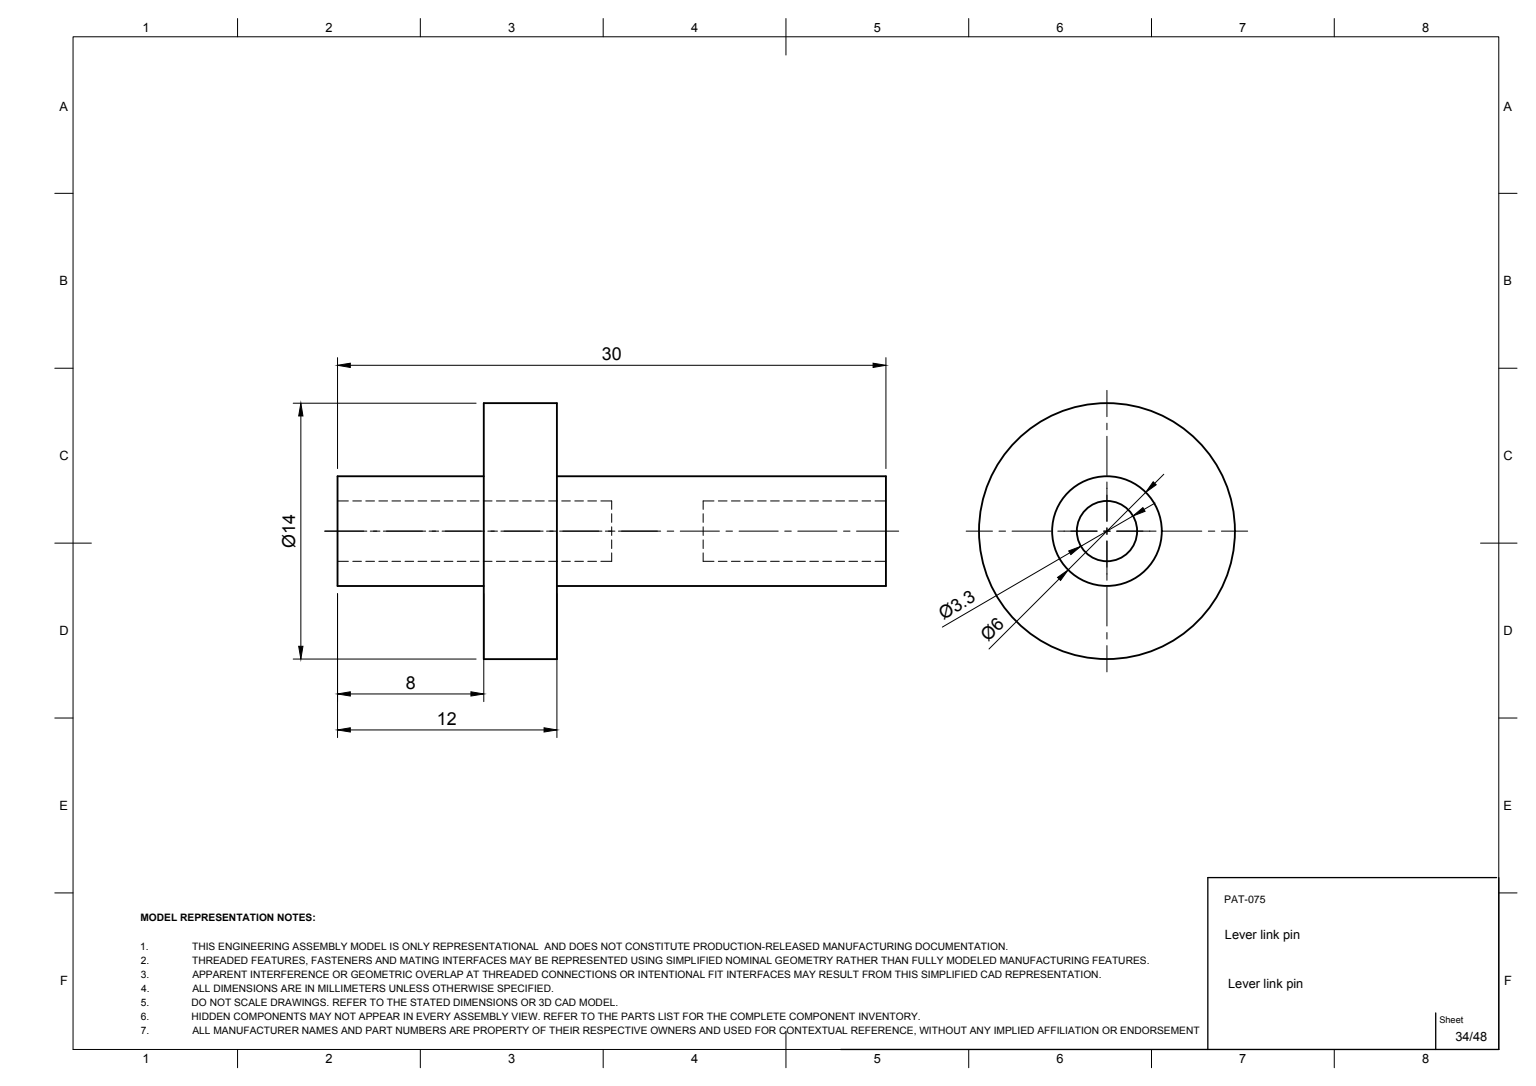
ISO-10303-21;
HEADER;
/* Generated by software containing ST-Developer
 * from STEP Tools, Inc. (www.steptools.com) 
 */

FILE_DESCRIPTION(
/* description */ ('Over-Centre Plunger Toggle Clamp on Slotted Fixture Frame'),
/* implementation_level */ '2;1');

FILE_NAME(
/* name */ 
'Lever link pin.step',
/* time_stamp */ '2026-10-28T03:23:24-07:00',
/* author */ (''),
/* organization */ (''),
/* preprocessor_version */ 'ST-DEVELOPER v20.2',
/* originating_system */ 'Autodesk Translation Framework v15.17.0.0',
/* authorisation */ '');

FILE_SCHEMA (('AUTOMOTIVE_DESIGN { 1 0 10303 214 3 1 1 }'));
ENDSEC;

DATA;
#10=MECHANICAL_DESIGN_GEOMETRIC_PRESENTATION_REPRESENTATION('',(#548),#15212);
#456=SHAPE_REPRESENTATION_RELATIONSHIP('SRR','None',#15433,#498);
#498=ADVANCED_BREP_SHAPE_REPRESENTATION('',(#597),#15195);
#548=STYLED_ITEM('',(#15719),#597);
#597=MANIFOLD_SOLID_BREP('Body1',#8282);
#753=FACE_BOUND('',#2075,.T.);
#754=FACE_BOUND('',#2077,.T.);
#755=FACE_BOUND('',#2082,.T.);
#756=FACE_BOUND('',#2084,.T.);
#1001=PLANE('',#9446);
#1002=PLANE('',#9450);
#1003=PLANE('',#9451);
#1004=PLANE('',#9454);
#1005=PLANE('',#9462);
#1006=PLANE('',#9463);
#1442=FACE_OUTER_BOUND('',#2070,.T.);
#1443=FACE_OUTER_BOUND('',#2071,.T.);
#1444=FACE_OUTER_BOUND('',#2072,.T.);
#1445=FACE_OUTER_BOUND('',#2073,.T.);
#1446=FACE_OUTER_BOUND('',#2074,.T.);
#1447=FACE_OUTER_BOUND('',#2076,.T.);
#1448=FACE_OUTER_BOUND('',#2078,.T.);
#1449=FACE_OUTER_BOUND('',#2079,.T.);
#1450=FACE_OUTER_BOUND('',#2080,.T.);
#1451=FACE_OUTER_BOUND('',#2081,.T.);
#1452=FACE_OUTER_BOUND('',#2083,.T.);
#2070=EDGE_LOOP('',(#7129,#7130,#7131,#7132));
#2071=EDGE_LOOP('',(#7133));
#2072=EDGE_LOOP('',(#7134,#7135,#7136,#7137));
#2073=EDGE_LOOP('',(#7138));
#2074=EDGE_LOOP('',(#7139));
#2075=EDGE_LOOP('',(#7140));
#2076=EDGE_LOOP('',(#7141));
#2077=EDGE_LOOP('',(#7142));
#2078=EDGE_LOOP('',(#7143,#7144,#7145,#7146));
#2079=EDGE_LOOP('',(#7147,#7148,#7149,#7150));
#2080=EDGE_LOOP('',(#7151,#7152,#7153,#7154));
#2081=EDGE_LOOP('',(#7155));
#2082=EDGE_LOOP('',(#7156));
#2083=EDGE_LOOP('',(#7157));
#2084=EDGE_LOOP('',(#7158));
#2704=LINE('',#14470,#3334);
#2705=LINE('',#14477,#3335);
#2706=LINE('',#14491,#3336);
#2707=LINE('',#14494,#3337);
#2708=LINE('',#14499,#3338);
#3334=VECTOR('',#11591,0.165);
#3335=VECTOR('',#11600,0.165);
#3336=VECTOR('',#11619,0.7);
#3337=VECTOR('',#11622,0.3);
#3338=VECTOR('',#11629,0.3);
#3774=CIRCLE('',#9444,0.165);
#3775=CIRCLE('',#9445,0.165);
#3776=CIRCLE('',#9448,0.165);
#3777=CIRCLE('',#9449,0.165);
#3778=CIRCLE('',#9452,0.7);
#3779=CIRCLE('',#9453,0.3);
#3780=CIRCLE('',#9455,0.7);
#3781=CIRCLE('',#9456,0.3);
#3782=CIRCLE('',#9459,0.3);
#3783=CIRCLE('',#9461,0.3);
#4386=VERTEX_POINT('',#14467);
#4387=VERTEX_POINT('',#14469);
#4388=VERTEX_POINT('',#14474);
#4389=VERTEX_POINT('',#14476);
#4390=VERTEX_POINT('',#14481);
#4391=VERTEX_POINT('',#14483);
#4392=VERTEX_POINT('',#14486);
#4393=VERTEX_POINT('',#14488);
#4394=VERTEX_POINT('',#14493);
#4395=VERTEX_POINT('',#14497);
#5325=EDGE_CURVE('',#4386,#4386,#3774,.T.);
#5326=EDGE_CURVE('',#4386,#4387,#2704,.T.);
#5327=EDGE_CURVE('',#4387,#4387,#3775,.T.);
#5328=EDGE_CURVE('',#4388,#4388,#3776,.T.);
#5329=EDGE_CURVE('',#4388,#4389,#2705,.T.);
#5330=EDGE_CURVE('',#4389,#4389,#3777,.T.);
#5331=EDGE_CURVE('',#4390,#4390,#3778,.T.);
#5332=EDGE_CURVE('',#4391,#4391,#3779,.T.);
#5333=EDGE_CURVE('',#4392,#4392,#3780,.T.);
#5334=EDGE_CURVE('',#4393,#4393,#3781,.T.);
#5335=EDGE_CURVE('',#4390,#4392,#2706,.T.);
#5336=EDGE_CURVE('',#4393,#4394,#2707,.T.);
#5337=EDGE_CURVE('',#4394,#4394,#3782,.T.);
#5338=EDGE_CURVE('',#4395,#4395,#3783,.T.);
#5339=EDGE_CURVE('',#4395,#4391,#2708,.T.);
#7129=ORIENTED_EDGE('',*,*,#5325,.F.);
#7130=ORIENTED_EDGE('',*,*,#5326,.T.);
#7131=ORIENTED_EDGE('',*,*,#5327,.F.);
#7132=ORIENTED_EDGE('',*,*,#5326,.F.);
#7133=ORIENTED_EDGE('',*,*,#5325,.T.);
#7134=ORIENTED_EDGE('',*,*,#5328,.F.);
#7135=ORIENTED_EDGE('',*,*,#5329,.T.);
#7136=ORIENTED_EDGE('',*,*,#5330,.T.);
#7137=ORIENTED_EDGE('',*,*,#5329,.F.);
#7138=ORIENTED_EDGE('',*,*,#5330,.F.);
#7139=ORIENTED_EDGE('',*,*,#5331,.T.);
#7140=ORIENTED_EDGE('',*,*,#5332,.F.);
#7141=ORIENTED_EDGE('',*,*,#5333,.F.);
#7142=ORIENTED_EDGE('',*,*,#5334,.F.);
#7143=ORIENTED_EDGE('',*,*,#5331,.F.);
#7144=ORIENTED_EDGE('',*,*,#5335,.T.);
#7145=ORIENTED_EDGE('',*,*,#5333,.T.);
#7146=ORIENTED_EDGE('',*,*,#5335,.F.);
#7147=ORIENTED_EDGE('',*,*,#5334,.T.);
#7148=ORIENTED_EDGE('',*,*,#5336,.T.);
#7149=ORIENTED_EDGE('',*,*,#5337,.T.);
#7150=ORIENTED_EDGE('',*,*,#5336,.F.);
#7151=ORIENTED_EDGE('',*,*,#5338,.F.);
#7152=ORIENTED_EDGE('',*,*,#5339,.T.);
#7153=ORIENTED_EDGE('',*,*,#5332,.T.);
#7154=ORIENTED_EDGE('',*,*,#5339,.F.);
#7155=ORIENTED_EDGE('',*,*,#5338,.T.);
#7156=ORIENTED_EDGE('',*,*,#5327,.T.);
#7157=ORIENTED_EDGE('',*,*,#5337,.F.);
#7158=ORIENTED_EDGE('',*,*,#5328,.T.);
#7724=CYLINDRICAL_SURFACE('',#9443,0.165);
#7725=CYLINDRICAL_SURFACE('',#9447,0.165);
#7726=CYLINDRICAL_SURFACE('',#9457,0.7);
#7727=CYLINDRICAL_SURFACE('',#9458,0.3);
#7728=CYLINDRICAL_SURFACE('',#9460,0.3);
#8114=ADVANCED_FACE('',(#1442),#7724,.F.);
#8115=ADVANCED_FACE('',(#1443),#1001,.T.);
#8116=ADVANCED_FACE('',(#1444),#7725,.F.);
#8117=ADVANCED_FACE('',(#1445),#1002,.F.);
#8118=ADVANCED_FACE('',(#1446,#753),#1003,.T.);
#8119=ADVANCED_FACE('',(#1447,#754),#1004,.F.);
#8120=ADVANCED_FACE('',(#1448),#7726,.T.);
#8121=ADVANCED_FACE('',(#1449),#7727,.T.);
#8122=ADVANCED_FACE('',(#1450),#7728,.T.);
#8123=ADVANCED_FACE('',(#1451,#755),#1005,.T.);
#8124=ADVANCED_FACE('',(#1452,#756),#1006,.F.);
#8282=CLOSED_SHELL('',(#8114,#8115,#8116,#8117,#8118,#8119,#8120,#8121,
#8122,#8123,#8124));
#9442=AXIS2_PLACEMENT_3D('',#14465,#11585,#11586);
#9443=AXIS2_PLACEMENT_3D('',#14466,#11587,#11588);
#9444=AXIS2_PLACEMENT_3D('',#14468,#11589,#11590);
#9445=AXIS2_PLACEMENT_3D('',#14471,#11592,#11593);
#9446=AXIS2_PLACEMENT_3D('',#14472,#11594,#11595);
#9447=AXIS2_PLACEMENT_3D('',#14473,#11596,#11597);
#9448=AXIS2_PLACEMENT_3D('',#14475,#11598,#11599);
#9449=AXIS2_PLACEMENT_3D('',#14478,#11601,#11602);
#9450=AXIS2_PLACEMENT_3D('',#14479,#11603,#11604);
#9451=AXIS2_PLACEMENT_3D('',#14480,#11605,#11606);
#9452=AXIS2_PLACEMENT_3D('',#14482,#11607,#11608);
#9453=AXIS2_PLACEMENT_3D('',#14484,#11609,#11610);
#9454=AXIS2_PLACEMENT_3D('',#14485,#11611,#11612);
#9455=AXIS2_PLACEMENT_3D('',#14487,#11613,#11614);
#9456=AXIS2_PLACEMENT_3D('',#14489,#11615,#11616);
#9457=AXIS2_PLACEMENT_3D('',#14490,#11617,#11618);
#9458=AXIS2_PLACEMENT_3D('',#14492,#11620,#11621);
#9459=AXIS2_PLACEMENT_3D('',#14495,#11623,#11624);
#9460=AXIS2_PLACEMENT_3D('',#14496,#11625,#11626);
#9461=AXIS2_PLACEMENT_3D('',#14498,#11627,#11628);
#9462=AXIS2_PLACEMENT_3D('',#14500,#11630,#11631);
#9463=AXIS2_PLACEMENT_3D('',#14501,#11632,#11633);
#11585=DIRECTION('axis',(0.,0.,1.));
#11586=DIRECTION('refdir',(1.,0.,0.));
#11587=DIRECTION('center_axis',(0.,1.,0.));
#11588=DIRECTION('ref_axis',(1.,0.,0.));
#11589=DIRECTION('center_axis',(0.,1.,0.));
#11590=DIRECTION('ref_axis',(1.,0.,0.));
#11591=DIRECTION('',(0.,1.,0.));
#11592=DIRECTION('center_axis',(0.,-1.,0.));
#11593=DIRECTION('ref_axis',(1.,0.,0.));
#11594=DIRECTION('center_axis',(0.,1.,0.));
#11595=DIRECTION('ref_axis',(1.,0.,0.));
#11596=DIRECTION('center_axis',(0.,1.,0.));
#11597=DIRECTION('ref_axis',(1.,0.,0.));
#11598=DIRECTION('center_axis',(0.,1.,0.));
#11599=DIRECTION('ref_axis',(1.,0.,0.));
#11600=DIRECTION('',(0.,1.,0.));
#11601=DIRECTION('center_axis',(0.,1.,0.));
#11602=DIRECTION('ref_axis',(1.,0.,0.));
#11603=DIRECTION('center_axis',(0.,1.,0.));
#11604=DIRECTION('ref_axis',(1.,0.,0.));
#11605=DIRECTION('center_axis',(0.,1.,0.));
#11606=DIRECTION('ref_axis',(1.,0.,0.));
#11607=DIRECTION('center_axis',(0.,1.,0.));
#11608=DIRECTION('ref_axis',(1.,0.,0.));
#11609=DIRECTION('center_axis',(0.,1.,0.));
#11610=DIRECTION('ref_axis',(1.,0.,0.));
#11611=DIRECTION('center_axis',(0.,1.,0.));
#11612=DIRECTION('ref_axis',(1.,0.,0.));
#11613=DIRECTION('center_axis',(0.,1.,0.));
#11614=DIRECTION('ref_axis',(1.,0.,0.));
#11615=DIRECTION('center_axis',(0.,-1.,0.));
#11616=DIRECTION('ref_axis',(1.,0.,0.));
#11617=DIRECTION('center_axis',(0.,1.,0.));
#11618=DIRECTION('ref_axis',(1.,0.,0.));
#11619=DIRECTION('',(0.,-1.,0.));
#11620=DIRECTION('center_axis',(0.,1.,0.));
#11621=DIRECTION('ref_axis',(1.,0.,0.));
#11622=DIRECTION('',(0.,-1.,0.));
#11623=DIRECTION('center_axis',(0.,1.,0.));
#11624=DIRECTION('ref_axis',(1.,0.,0.));
#11625=DIRECTION('center_axis',(0.,1.,0.));
#11626=DIRECTION('ref_axis',(1.,0.,0.));
#11627=DIRECTION('center_axis',(0.,1.,0.));
#11628=DIRECTION('ref_axis',(1.,0.,0.));
#11629=DIRECTION('',(0.,-1.,0.));
#11630=DIRECTION('center_axis',(0.,1.,0.));
#11631=DIRECTION('ref_axis',(1.,0.,0.));
#11632=DIRECTION('center_axis',(0.,1.,0.));
#11633=DIRECTION('ref_axis',(1.,0.,0.));
#14465=CARTESIAN_POINT('',(0.,0.,0.));
#14466=CARTESIAN_POINT('Origin',(-2.82632109303527,-4.2,8.79263101785268));
#14467=CARTESIAN_POINT('',(-2.99132109303527,-4.2,8.79263101785268));
#14468=CARTESIAN_POINT('Origin',(-2.82632109303527,-4.2,8.79263101785268));
#14469=CARTESIAN_POINT('',(-2.99132109303527,-2.7,8.79263101785268));
#14470=CARTESIAN_POINT('',(-2.99132109303527,-4.2,8.79263101785268));
#14471=CARTESIAN_POINT('Origin',(-2.82632109303527,-2.7,8.79263101785268));
#14472=CARTESIAN_POINT('Origin',(-2.82632109303527,-4.2,8.79263101785268));
#14473=CARTESIAN_POINT('Origin',(-2.82632109303527,-5.8,8.79263101785268));
#14474=CARTESIAN_POINT('',(-2.99132109303527,-5.7,8.79263101785268));
#14475=CARTESIAN_POINT('Origin',(-2.82632109303527,-5.7,8.79263101785268));
#14476=CARTESIAN_POINT('',(-2.99132109303527,-4.7,8.79263101785268));
#14477=CARTESIAN_POINT('',(-2.99132109303527,-5.8,8.79263101785268));
#14478=CARTESIAN_POINT('Origin',(-2.82632109303527,-4.7,8.79263101785268));
#14479=CARTESIAN_POINT('Origin',(-2.82632109303527,-4.7,8.79263101785268));
#14480=CARTESIAN_POINT('Origin',(-2.82632109303527,-3.5,8.79263101785268));
#14481=CARTESIAN_POINT('',(-3.52632109303527,-3.5,8.79263101785268));
#14482=CARTESIAN_POINT('Origin',(-2.82632109303527,-3.5,8.79263101785268));
#14483=CARTESIAN_POINT('',(-3.12632109303527,-3.5,8.79263101785268));
#14484=CARTESIAN_POINT('Origin',(-2.82632109303527,-3.5,8.79263101785268));
#14485=CARTESIAN_POINT('Origin',(-2.82632109303527,-3.9,8.79263101785268));
#14486=CARTESIAN_POINT('',(-3.52632109303527,-3.9,8.79263101785268));
#14487=CARTESIAN_POINT('Origin',(-2.82632109303527,-3.9,8.79263101785268));
#14488=CARTESIAN_POINT('',(-3.12632109303527,-3.9,8.79263101785268));
#14489=CARTESIAN_POINT('Origin',(-2.82632109303527,-3.9,8.79263101785268));
#14490=CARTESIAN_POINT('Origin',(-2.82632109303527,-3.9,8.79263101785268));
#14491=CARTESIAN_POINT('',(-3.52632109303527,-3.9,8.79263101785268));
#14492=CARTESIAN_POINT('Origin',(-2.82632109303527,-5.7,8.79263101785268));
#14493=CARTESIAN_POINT('',(-3.12632109303527,-5.7,8.79263101785268));
#14494=CARTESIAN_POINT('',(-3.12632109303527,-5.7,8.79263101785268));
#14495=CARTESIAN_POINT('Origin',(-2.82632109303527,-5.7,8.79263101785268));
#14496=CARTESIAN_POINT('Origin',(-2.82632109303527,-5.7,8.79263101785268));
#14497=CARTESIAN_POINT('',(-3.12632109303527,-2.7,8.79263101785268));
#14498=CARTESIAN_POINT('Origin',(-2.82632109303527,-2.7,8.79263101785268));
#14499=CARTESIAN_POINT('',(-3.12632109303527,-5.7,8.79263101785268));
#14500=CARTESIAN_POINT('Origin',(-2.82632109303527,-2.7,8.79263101785268));
#14501=CARTESIAN_POINT('Origin',(-2.82632109303527,-5.7,8.79263101785268));
#15145=UNCERTAINTY_MEASURE_WITH_UNIT(LENGTH_MEASURE(0.001),#15213,
'DISTANCE_ACCURACY_VALUE',
'Maximum model space distance between geometric entities at asserted c
onnectivities');
#15162=UNCERTAINTY_MEASURE_WITH_UNIT(LENGTH_MEASURE(0.001),#15213,
'DISTANCE_ACCURACY_VALUE',
'Maximum model space distance between geometric entities at asserted c
onnectivities');
#15195=(
GEOMETRIC_REPRESENTATION_CONTEXT(3)
GLOBAL_UNCERTAINTY_ASSIGNED_CONTEXT((#15145))
GLOBAL_UNIT_ASSIGNED_CONTEXT((#15213,#15215,#15216))
REPRESENTATION_CONTEXT('','3D')
);
#15212=(
GEOMETRIC_REPRESENTATION_CONTEXT(3)
GLOBAL_UNCERTAINTY_ASSIGNED_CONTEXT((#15162))
GLOBAL_UNIT_ASSIGNED_CONTEXT((#15213,#15215,#15216))
REPRESENTATION_CONTEXT('','3D')
);
#15213=(
LENGTH_UNIT()
NAMED_UNIT(*)
SI_UNIT(.CENTI.,.METRE.)
);
#15215=(
NAMED_UNIT(*)
PLANE_ANGLE_UNIT()
SI_UNIT($,.RADIAN.)
);
#15216=(
NAMED_UNIT(*)
SI_UNIT($,.STERADIAN.)
SOLID_ANGLE_UNIT()
);
#15249=SHAPE_DEFINITION_REPRESENTATION(#15305,#15433);
#15305=PRODUCT_DEFINITION_SHAPE('',$,#15483);
#15433=SHAPE_REPRESENTATION('',(#9442),#15195);
#15450=PRODUCT_DEFINITION_CONTEXT('part definition',#15599,'design');
#15483=PRODUCT_DEFINITION('Lever link pin','Lever link pin',#15532,#15450);
#15532=PRODUCT_DEFINITION_FORMATION('',$,#15633);
#15599=APPLICATION_CONTEXT(
'Core Data for Automotive Mechanical Design Process');
#15600=PRODUCT_CONTEXT('part definition',#15599,'mechanical');
#15633=PRODUCT('Lever link pin','Lever link pin','Lever link pin',(#15600));
#15713=COLOUR_RGB('Grey',0.48,0.52,0.57);
#15714=FILL_AREA_STYLE_COLOUR('',#15713);
#15715=FILL_AREA_STYLE('',(#15714));
#15716=SURFACE_STYLE_FILL_AREA(#15715);
#15717=SURFACE_SIDE_STYLE('',(#15716));
#15718=SURFACE_STYLE_USAGE(.BOTH.,#15717);
#15719=PRESENTATION_STYLE_ASSIGNMENT((#15718));
ENDSEC;
END-ISO-10303-21;
